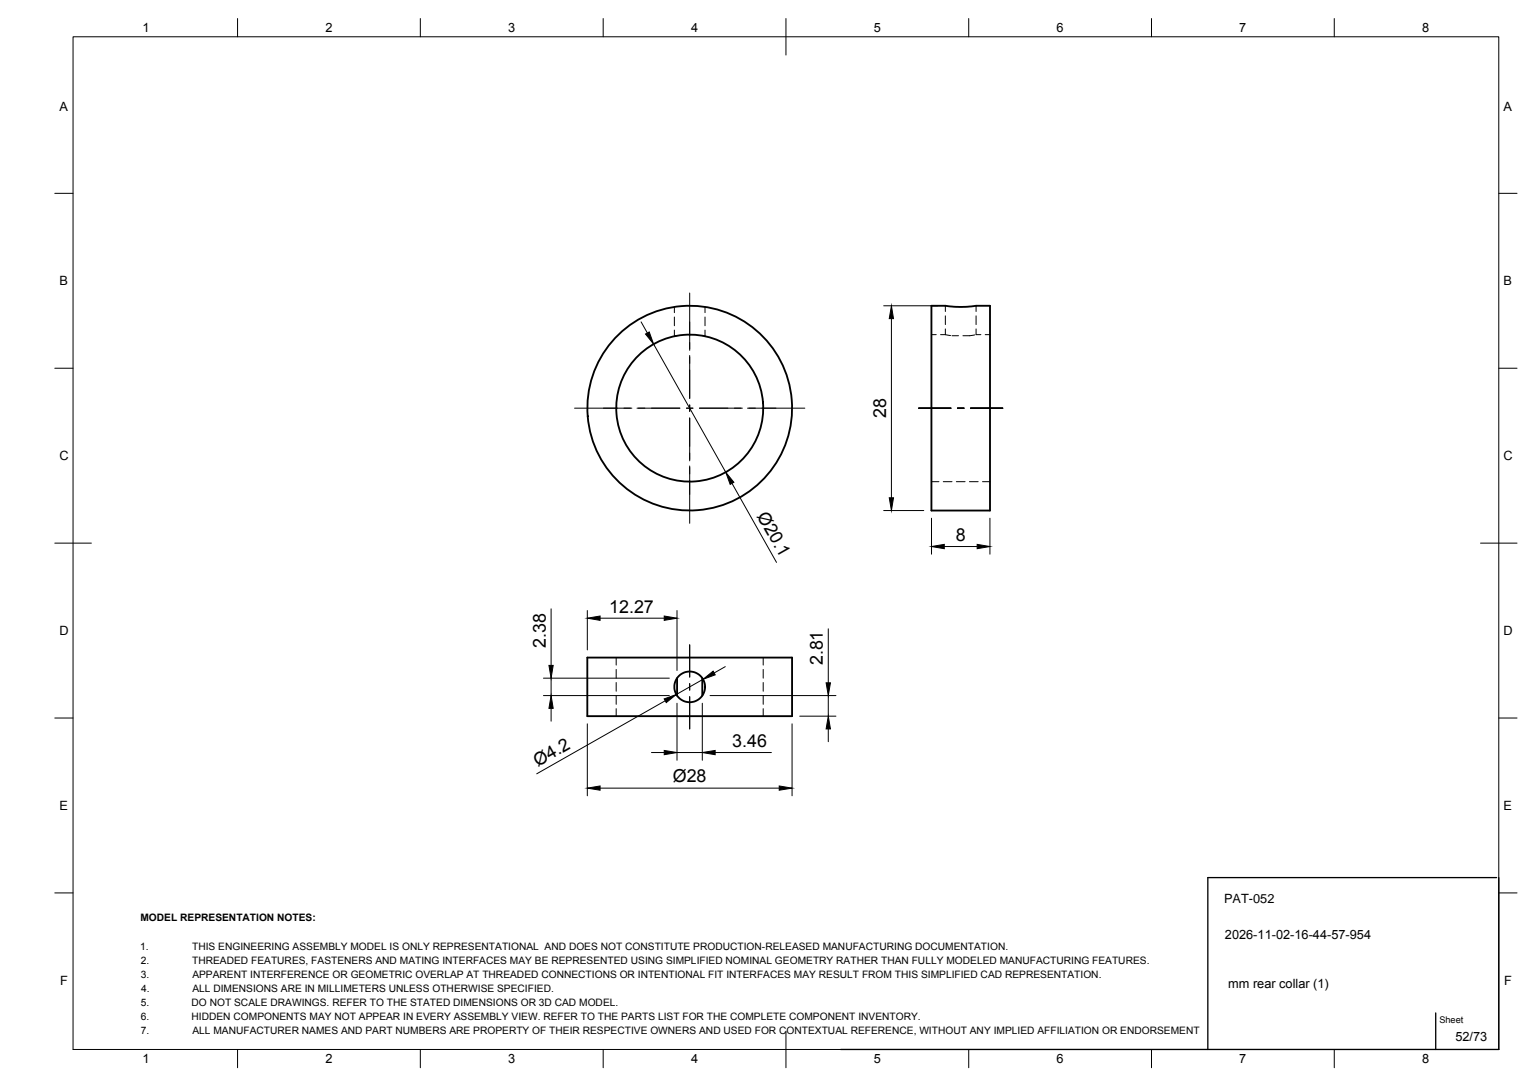
ISO-10303-21;
HEADER;
/* Generated by software containing ST-Developer
 * from STEP Tools, Inc. (www.steptools.com) 
 */

FILE_DESCRIPTION(
/* description */ ('Hand-crank gear train demonstrator'),
/* implementation_level */ '2;1');

FILE_NAME(
/* name */ 'mm rear collar (1).step',
/* time_stamp */ '2026-10-28T03:22:13-07:00',
/* author */ (''),
/* organization */ (''),
/* preprocessor_version */ 'ST-DEVELOPER v20.2',
/* originating_system */ 'Autodesk Translation Framework v15.17.0.0',
/* authorisation */ '');

FILE_SCHEMA (('AUTOMOTIVE_DESIGN { 1 0 10303 214 3 1 1 }'));
ENDSEC;

DATA;
#10=MECHANICAL_DESIGN_GEOMETRIC_PRESENTATION_REPRESENTATION('',(#1246),#62758);
#895=B_SPLINE_CURVE_WITH_KNOTS('',3,(#26487,#26488,#26489,#26490,#26491,
#26492,#26493,#26494,#26495,#26496,#26497,#26498,#26499,#26500),
 .UNSPECIFIED.,.F.,.F.,(4,2,2,2,2,2,4),(0.75600573798703,0.793568827564647,
0.872922520054202,0.952276212543757,1.03162990503331,1.11098359752287,1.14854668710048),
 .UNSPECIFIED.);
#896=B_SPLINE_CURVE_WITH_KNOTS('',3,(#26506,#26507,#26508,#26509,#26510,
#26511,#26512,#26513,#26514,#26515,#26516,#26517,#26518,#26519,#26520,#26521,
#26522,#26523),.UNSPECIFIED.,.F.,.F.,(4,2,2,2,2,2,2,2,4),(0.,0.0792334805614372,
0.158466961122874,0.237699060165217,0.31693115920756,0.396163258249903,
0.475395357292246,0.554628837853683,0.63386231841512),.UNSPECIFIED.);
#897=B_SPLINE_CURVE_WITH_KNOTS('',3,(#26524,#26525,#26526,#26527,#26528,
#26529,#26530,#26531,#26532,#26533,#26534,#26535,#26536,#26537,#26538,#26539,
#26540,#26541),.UNSPECIFIED.,.F.,.F.,(4,2,2,2,2,2,2,2,4),(0.63386231841512,
0.713095798976557,0.792329279537994,0.871561378580337,0.95079347762268,
1.03002557666502,1.10925767570737,1.1884911562688,1.26772463683024),
 .UNSPECIFIED.);
#898=B_SPLINE_CURVE_WITH_KNOTS('',3,(#26544,#26545,#26546,#26547,#26548,
#26549,#26550,#26551,#26552,#26553,#26554,#26555,#26556,#26557),
 .UNSPECIFIED.,.F.,.F.,(4,2,2,2,2,2,4),(0.121154929624526,0.158718019202142,
0.238071711691697,0.317425404181252,0.396779096670807,0.476132789160362,
0.513695878737979),.UNSPECIFIED.);
#1103=SHAPE_REPRESENTATION_RELATIONSHIP('SRR','None',#63079,#1167);
#1167=ADVANCED_BREP_SHAPE_REPRESENTATION('',(#1321),#62733);
#1246=STYLED_ITEM('',(#63448),#1321);
#1321=MANIFOLD_SOLID_BREP('Body1',#16430);
#1580=FACE_BOUND('',#3832,.T.);
#1581=FACE_BOUND('',#3834,.T.);
#1582=FACE_BOUND('',#3836,.T.);
#1583=FACE_BOUND('',#3838,.T.);
#1951=PLANE('',#18180);
#1952=PLANE('',#18185);
#1953=PLANE('',#18192);
#1954=PLANE('',#18193);
#2654=FACE_OUTER_BOUND('',#3828,.T.);
#2655=FACE_OUTER_BOUND('',#3829,.T.);
#2656=FACE_OUTER_BOUND('',#3830,.T.);
#2657=FACE_OUTER_BOUND('',#3831,.T.);
#2658=FACE_OUTER_BOUND('',#3833,.T.);
#2659=FACE_OUTER_BOUND('',#3835,.T.);
#2660=FACE_OUTER_BOUND('',#3837,.T.);
#3828=EDGE_LOOP('',(#13095,#13096));
#3829=EDGE_LOOP('',(#13097,#13098,#13099,#13100,#13101,#13102,#13103,#13104,
#13105));
#3830=EDGE_LOOP('',(#13106,#13107,#13108));
#3831=EDGE_LOOP('',(#13109,#13110,#13111,#13112));
#3832=EDGE_LOOP('',(#13113,#13114,#13115,#13116));
#3833=EDGE_LOOP('',(#13117,#13118,#13119,#13120));
#3834=EDGE_LOOP('',(#13121,#13122));
#3835=EDGE_LOOP('',(#13123));
#3836=EDGE_LOOP('',(#13124));
#3837=EDGE_LOOP('',(#13125));
#3838=EDGE_LOOP('',(#13126));
#4948=LINE('',#26483,#6080);
#4949=LINE('',#26504,#6081);
#4950=LINE('',#26559,#6082);
#4951=LINE('',#26564,#6083);
#4952=LINE('',#26570,#6084);
#6080=VECTOR('',#21539,1.);
#6081=VECTOR('',#21546,0.21);
#6082=VECTOR('',#21551,1.);
#6083=VECTOR('',#21556,1.005);
#6084=VECTOR('',#21563,1.4);
#6982=CIRCLE('',#18181,0.21);
#6983=CIRCLE('',#18183,0.21);
#6984=CIRCLE('',#18184,0.21);
#6985=CIRCLE('',#18187,1.005);
#6986=CIRCLE('',#18188,1.005);
#6987=CIRCLE('',#18190,1.4);
#6988=CIRCLE('',#18191,1.4);
#7979=VERTEX_POINT('',#26481);
#7980=VERTEX_POINT('',#26482);
#7981=VERTEX_POINT('',#26486);
#7982=VERTEX_POINT('',#26501);
#7983=VERTEX_POINT('',#26503);
#7984=VERTEX_POINT('',#26505);
#7985=VERTEX_POINT('',#26542);
#7986=VERTEX_POINT('',#26561);
#7987=VERTEX_POINT('',#26563);
#7988=VERTEX_POINT('',#26567);
#7989=VERTEX_POINT('',#26569);
#9799=EDGE_CURVE('',#7979,#7980,#4948,.T.);
#9800=EDGE_CURVE('',#7979,#7980,#6982,.T.);
#9801=EDGE_CURVE('',#7981,#7979,#895,.T.);
#9802=EDGE_CURVE('',#7982,#7981,#6983,.T.);
#9803=EDGE_CURVE('',#7982,#7983,#4949,.T.);
#9804=EDGE_CURVE('',#7984,#7983,#896,.T.);
#9805=EDGE_CURVE('',#7983,#7984,#897,.T.);
#9806=EDGE_CURVE('',#7985,#7982,#6984,.T.);
#9807=EDGE_CURVE('',#7980,#7985,#898,.T.);
#9808=EDGE_CURVE('',#7985,#7981,#4950,.T.);
#9809=EDGE_CURVE('',#7986,#7986,#6985,.T.);
#9810=EDGE_CURVE('',#7986,#7987,#4951,.T.);
#9811=EDGE_CURVE('',#7987,#7987,#6986,.T.);
#9812=EDGE_CURVE('',#7988,#7988,#6987,.T.);
#9813=EDGE_CURVE('',#7988,#7989,#4952,.T.);
#9814=EDGE_CURVE('',#7989,#7989,#6988,.T.);
#13095=ORIENTED_EDGE('',*,*,#9799,.F.);
#13096=ORIENTED_EDGE('',*,*,#9800,.T.);
#13097=ORIENTED_EDGE('',*,*,#9801,.F.);
#13098=ORIENTED_EDGE('',*,*,#9802,.F.);
#13099=ORIENTED_EDGE('',*,*,#9803,.T.);
#13100=ORIENTED_EDGE('',*,*,#9804,.F.);
#13101=ORIENTED_EDGE('',*,*,#9805,.F.);
#13102=ORIENTED_EDGE('',*,*,#9803,.F.);
#13103=ORIENTED_EDGE('',*,*,#9806,.F.);
#13104=ORIENTED_EDGE('',*,*,#9807,.F.);
#13105=ORIENTED_EDGE('',*,*,#9800,.F.);
#13106=ORIENTED_EDGE('',*,*,#9808,.F.);
#13107=ORIENTED_EDGE('',*,*,#9806,.T.);
#13108=ORIENTED_EDGE('',*,*,#9802,.T.);
#13109=ORIENTED_EDGE('',*,*,#9809,.F.);
#13110=ORIENTED_EDGE('',*,*,#9810,.T.);
#13111=ORIENTED_EDGE('',*,*,#9811,.T.);
#13112=ORIENTED_EDGE('',*,*,#9810,.F.);
#13113=ORIENTED_EDGE('',*,*,#9807,.T.);
#13114=ORIENTED_EDGE('',*,*,#9808,.T.);
#13115=ORIENTED_EDGE('',*,*,#9801,.T.);
#13116=ORIENTED_EDGE('',*,*,#9799,.T.);
#13117=ORIENTED_EDGE('',*,*,#9812,.F.);
#13118=ORIENTED_EDGE('',*,*,#9813,.T.);
#13119=ORIENTED_EDGE('',*,*,#9814,.T.);
#13120=ORIENTED_EDGE('',*,*,#9813,.F.);
#13121=ORIENTED_EDGE('',*,*,#9804,.T.);
#13122=ORIENTED_EDGE('',*,*,#9805,.T.);
#13123=ORIENTED_EDGE('',*,*,#9812,.T.);
#13124=ORIENTED_EDGE('',*,*,#9809,.T.);
#13125=ORIENTED_EDGE('',*,*,#9814,.F.);
#13126=ORIENTED_EDGE('',*,*,#9811,.F.);
#15326=CYLINDRICAL_SURFACE('',#18182,0.21);
#15327=CYLINDRICAL_SURFACE('',#18186,1.005);
#15328=CYLINDRICAL_SURFACE('',#18189,1.4);
#15964=ADVANCED_FACE('',(#2654),#1951,.T.);
#15965=ADVANCED_FACE('',(#2655),#15326,.F.);
#15966=ADVANCED_FACE('',(#2656),#1952,.T.);
#15967=ADVANCED_FACE('',(#2657,#1580),#15327,.F.);
#15968=ADVANCED_FACE('',(#2658,#1581),#15328,.T.);
#15969=ADVANCED_FACE('',(#2659,#1582),#1953,.T.);
#15970=ADVANCED_FACE('',(#2660,#1583),#1954,.F.);
#16430=CLOSED_SHELL('',(#15964,#15965,#15966,#15967,#15968,#15969,#15970));
#18179=AXIS2_PLACEMENT_3D('',#26479,#21535,#21536);
#18180=AXIS2_PLACEMENT_3D('',#26480,#21537,#21538);
#18181=AXIS2_PLACEMENT_3D('',#26484,#21540,#21541);
#18182=AXIS2_PLACEMENT_3D('',#26485,#21542,#21543);
#18183=AXIS2_PLACEMENT_3D('',#26502,#21544,#21545);
#18184=AXIS2_PLACEMENT_3D('',#26543,#21547,#21548);
#18185=AXIS2_PLACEMENT_3D('',#26558,#21549,#21550);
#18186=AXIS2_PLACEMENT_3D('',#26560,#21552,#21553);
#18187=AXIS2_PLACEMENT_3D('',#26562,#21554,#21555);
#18188=AXIS2_PLACEMENT_3D('',#26565,#21557,#21558);
#18189=AXIS2_PLACEMENT_3D('',#26566,#21559,#21560);
#18190=AXIS2_PLACEMENT_3D('',#26568,#21561,#21562);
#18191=AXIS2_PLACEMENT_3D('',#26571,#21564,#21565);
#18192=AXIS2_PLACEMENT_3D('',#26572,#21566,#21567);
#18193=AXIS2_PLACEMENT_3D('',#26573,#21568,#21569);
#21535=DIRECTION('axis',(0.,0.,1.));
#21536=DIRECTION('refdir',(1.,0.,0.));
#21537=DIRECTION('center_axis',(0.,0.,1.));
#21538=DIRECTION('ref_axis',(1.,0.,0.));
#21539=DIRECTION('',(0.,1.,0.));
#21540=DIRECTION('center_axis',(0.,0.,1.));
#21541=DIRECTION('ref_axis',(1.,0.,0.));
#21542=DIRECTION('center_axis',(0.,0.,1.));
#21543=DIRECTION('ref_axis',(1.,0.,0.));
#21544=DIRECTION('center_axis',(0.,0.,1.));
#21545=DIRECTION('ref_axis',(1.,0.,0.));
#21546=DIRECTION('',(0.,0.,1.));
#21547=DIRECTION('center_axis',(0.,0.,1.));
#21548=DIRECTION('ref_axis',(1.,0.,0.));
#21549=DIRECTION('center_axis',(0.,0.,1.));
#21550=DIRECTION('ref_axis',(1.,0.,0.));
#21551=DIRECTION('',(0.,-1.,0.));
#21552=DIRECTION('center_axis',(0.,1.,0.));
#21553=DIRECTION('ref_axis',(1.,0.,0.));
#21554=DIRECTION('center_axis',(0.,-1.,0.));
#21555=DIRECTION('ref_axis',(1.,0.,0.));
#21556=DIRECTION('',(0.,-1.,0.));
#21557=DIRECTION('center_axis',(0.,-1.,0.));
#21558=DIRECTION('ref_axis',(1.,0.,0.));
#21559=DIRECTION('center_axis',(0.,1.,0.));
#21560=DIRECTION('ref_axis',(1.,0.,0.));
#21561=DIRECTION('center_axis',(0.,1.,0.));
#21562=DIRECTION('ref_axis',(1.,0.,0.));
#21563=DIRECTION('',(0.,-1.,0.));
#21564=DIRECTION('center_axis',(0.,1.,0.));
#21565=DIRECTION('ref_axis',(1.,0.,0.));
#21566=DIRECTION('center_axis',(0.,1.,0.));
#21567=DIRECTION('ref_axis',(1.,0.,0.));
#21568=DIRECTION('center_axis',(0.,1.,0.));
#21569=DIRECTION('ref_axis',(1.,0.,0.));
#26479=CARTESIAN_POINT('',(0.,0.,0.));
#26480=CARTESIAN_POINT('Origin',(6.,-3.2,9.99));
#26481=CARTESIAN_POINT('',(6.17298843892005,-3.31905880899792,9.99));
#26482=CARTESIAN_POINT('',(6.17298843892005,-3.08094119100208,9.99));
#26483=CARTESIAN_POINT('',(6.17298843892005,-3.6,9.99));
#26484=CARTESIAN_POINT('Origin',(6.,-3.2,9.99));
#26485=CARTESIAN_POINT('Origin',(6.,-3.2,9.99));
#26486=CARTESIAN_POINT('',(5.82701156107995,-3.31905880899792,9.99));
#26487=CARTESIAN_POINT('Ctrl Pts',(5.82701156107995,-3.31905880899792,9.99));
#26488=CARTESIAN_POINT('Ctrl Pts',(5.83440513468869,-3.3298014223953,9.99129192197638));
#26489=CARTESIAN_POINT('Ctrl Pts',(5.8427028612744,-3.33968770937275,9.99265394943905));
#26490=CARTESIAN_POINT('Ctrl Pts',(5.87010792615492,-3.36709277425327,9.9967480843909));
#26491=CARTESIAN_POINT('Ctrl Pts',(5.89366983224072,-3.38324205633295,9.99969589327638));
#26492=CARTESIAN_POINT('Ctrl Pts',(5.94538709536759,-3.40469779396491,10.0038502947236));
#26493=CARTESIAN_POINT('Ctrl Pts',(5.97354876917015,-3.41,10.005));
#26494=CARTESIAN_POINT('Ctrl Pts',(6.02645123082985,-3.41,10.005));
#26495=CARTESIAN_POINT('Ctrl Pts',(6.05461290463241,-3.40469779396491,10.0038502947236));
#26496=CARTESIAN_POINT('Ctrl Pts',(6.10633016775928,-3.38324205633295,9.99969589327638));
#26497=CARTESIAN_POINT('Ctrl Pts',(6.12989207384508,-3.36709277425327,9.9967480843909));
#26498=CARTESIAN_POINT('Ctrl Pts',(6.1572971387256,-3.33968770937275,9.99265394943905));
#26499=CARTESIAN_POINT('Ctrl Pts',(6.16559486531131,-3.3298014223953,9.99129192197638));
#26500=CARTESIAN_POINT('Ctrl Pts',(6.17298843892005,-3.31905880899792,9.99));
#26501=CARTESIAN_POINT('',(5.79,-3.2,9.99));
#26502=CARTESIAN_POINT('Origin',(6.,-3.2,9.99));
#26503=CARTESIAN_POINT('',(5.79,-3.2,10.38416039533));
#26504=CARTESIAN_POINT('',(5.79,-3.2,9.99));
#26505=CARTESIAN_POINT('',(6.21,-3.2,10.38416039533));
#26506=CARTESIAN_POINT('Ctrl Pts',(6.21,-3.2,10.38416039533));
#26507=CARTESIAN_POINT('Ctrl Pts',(6.21,-3.22641116018715,10.38416039533));
#26508=CARTESIAN_POINT('Ctrl Pts',(6.20471354911189,-3.2545550596171,10.3849944296993));
#26509=CARTESIAN_POINT('Ctrl Pts',(6.18326999585849,-3.30628264999174,10.3879947099895));
#26510=CARTESIAN_POINT('Ctrl Pts',(6.16711503760643,-3.32986981049192,10.3901162943626));
#26511=CARTESIAN_POINT('Ctrl Pts',(6.12987013519678,-3.36711471290157,10.394089123191));
#26512=CARTESIAN_POINT('Ctrl Pts',(6.10628283459019,-3.38326992585508,10.3962002442067));
#26513=CARTESIAN_POINT('Ctrl Pts',(6.05455476560391,-3.40471366447292,10.3991765222353));
#26514=CARTESIAN_POINT('Ctrl Pts',(6.02641069968078,-3.41,10.4));
#26515=CARTESIAN_POINT('Ctrl Pts',(5.97358930031922,-3.41,10.4));
#26516=CARTESIAN_POINT('Ctrl Pts',(5.94544523439609,-3.40471366447292,10.3991765222353));
#26517=CARTESIAN_POINT('Ctrl Pts',(5.89371716540981,-3.38326992585508,10.3962002442067));
#26518=CARTESIAN_POINT('Ctrl Pts',(5.87012986480322,-3.36711471290157,10.394089123191));
#26519=CARTESIAN_POINT('Ctrl Pts',(5.83288496239357,-3.32986981049192,10.3901162943626));
#26520=CARTESIAN_POINT('Ctrl Pts',(5.81673000414151,-3.30628264999174,10.3879947099895));
#26521=CARTESIAN_POINT('Ctrl Pts',(5.79528645088811,-3.2545550596171,10.3849944296993));
#26522=CARTESIAN_POINT('Ctrl Pts',(5.79,-3.22641116018715,10.38416039533));
#26523=CARTESIAN_POINT('Ctrl Pts',(5.79,-3.2,10.38416039533));
#26524=CARTESIAN_POINT('Ctrl Pts',(5.79,-3.2,10.38416039533));
#26525=CARTESIAN_POINT('Ctrl Pts',(5.79,-3.17358883981285,10.38416039533));
#26526=CARTESIAN_POINT('Ctrl Pts',(5.79528645088811,-3.1454449403829,10.3849944296993));
#26527=CARTESIAN_POINT('Ctrl Pts',(5.81673000414151,-3.09371735000826,10.3879947099895));
#26528=CARTESIAN_POINT('Ctrl Pts',(5.83288496239357,-3.07013018950808,10.3901162943626));
#26529=CARTESIAN_POINT('Ctrl Pts',(5.87012986480322,-3.03288528709844,10.394089123191));
#26530=CARTESIAN_POINT('Ctrl Pts',(5.89371716540981,-3.01673007414492,10.3962002442067));
#26531=CARTESIAN_POINT('Ctrl Pts',(5.94544523439609,-2.99528633552708,10.3991765222353));
#26532=CARTESIAN_POINT('Ctrl Pts',(5.97358930031922,-2.99,10.4));
#26533=CARTESIAN_POINT('Ctrl Pts',(6.02641069968078,-2.99,10.4));
#26534=CARTESIAN_POINT('Ctrl Pts',(6.05455476560391,-2.99528633552708,10.3991765222353));
#26535=CARTESIAN_POINT('Ctrl Pts',(6.10628283459019,-3.01673007414492,10.3962002442067));
#26536=CARTESIAN_POINT('Ctrl Pts',(6.12987013519678,-3.03288528709844,10.394089123191));
#26537=CARTESIAN_POINT('Ctrl Pts',(6.16711503760643,-3.07013018950808,10.3901162943626));
#26538=CARTESIAN_POINT('Ctrl Pts',(6.18326999585849,-3.09371735000826,10.3879947099895));
#26539=CARTESIAN_POINT('Ctrl Pts',(6.20471354911189,-3.1454449403829,10.3849944296993));
#26540=CARTESIAN_POINT('Ctrl Pts',(6.21,-3.17358883981285,10.38416039533));
#26541=CARTESIAN_POINT('Ctrl Pts',(6.21,-3.2,10.38416039533));
#26542=CARTESIAN_POINT('',(5.82701156107995,-3.08094119100208,9.99));
#26543=CARTESIAN_POINT('Origin',(6.,-3.2,9.99));
#26544=CARTESIAN_POINT('Ctrl Pts',(6.17298843892005,-3.08094119100208,9.99));
#26545=CARTESIAN_POINT('Ctrl Pts',(6.16559486531131,-3.0701985776047,9.99129192197638));
#26546=CARTESIAN_POINT('Ctrl Pts',(6.15729713872561,-3.06031229062725,9.99265394943905));
#26547=CARTESIAN_POINT('Ctrl Pts',(6.12989207384508,-3.03290722574673,9.9967480843909));
#26548=CARTESIAN_POINT('Ctrl Pts',(6.10633016775929,-3.01675794366705,9.99969589327638));
#26549=CARTESIAN_POINT('Ctrl Pts',(6.05461290463241,-2.99530220603509,10.0038502947236));
#26550=CARTESIAN_POINT('Ctrl Pts',(6.02645123082985,-2.99,10.005));
#26551=CARTESIAN_POINT('Ctrl Pts',(5.97354876917015,-2.99,10.005));
#26552=CARTESIAN_POINT('Ctrl Pts',(5.94538709536759,-2.99530220603509,10.0038502947236));
#26553=CARTESIAN_POINT('Ctrl Pts',(5.89366983224072,-3.01675794366705,9.99969589327638));
#26554=CARTESIAN_POINT('Ctrl Pts',(5.87010792615492,-3.03290722574673,9.9967480843909));
#26555=CARTESIAN_POINT('Ctrl Pts',(5.8427028612744,-3.06031229062725,9.99265394943905));
#26556=CARTESIAN_POINT('Ctrl Pts',(5.83440513468869,-3.0701985776047,9.99129192197638));
#26557=CARTESIAN_POINT('Ctrl Pts',(5.82701156107995,-3.08094119100208,9.99));
#26558=CARTESIAN_POINT('Origin',(6.,-3.2,9.99));
#26559=CARTESIAN_POINT('',(5.82701156107995,-3.6,9.99));
#26560=CARTESIAN_POINT('Origin',(6.,-3.6,9.));
#26561=CARTESIAN_POINT('',(4.995,-2.8,9.));
#26562=CARTESIAN_POINT('Origin',(6.,-2.8,9.));
#26563=CARTESIAN_POINT('',(4.995,-3.6,9.));
#26564=CARTESIAN_POINT('',(4.995,-3.6,9.));
#26565=CARTESIAN_POINT('Origin',(6.,-3.6,9.));
#26566=CARTESIAN_POINT('Origin',(6.,-3.6,9.));
#26567=CARTESIAN_POINT('',(4.6,-2.8,9.));
#26568=CARTESIAN_POINT('Origin',(6.,-2.8,9.));
#26569=CARTESIAN_POINT('',(4.6,-3.6,9.));
#26570=CARTESIAN_POINT('',(4.6,-3.6,9.));
#26571=CARTESIAN_POINT('Origin',(6.,-3.6,9.));
#26572=CARTESIAN_POINT('Origin',(6.,-2.8,9.));
#26573=CARTESIAN_POINT('Origin',(6.,-3.6,9.));
#62659=UNCERTAINTY_MEASURE_WITH_UNIT(LENGTH_MEASURE(0.001),#62759,
'DISTANCE_ACCURACY_VALUE',
'Maximum model space distance between geometric entities at asserted c
onnectivities');
#62684=UNCERTAINTY_MEASURE_WITH_UNIT(LENGTH_MEASURE(0.001),#62759,
'DISTANCE_ACCURACY_VALUE',
'Maximum model space distance between geometric entities at asserted c
onnectivities');
#62733=(
GEOMETRIC_REPRESENTATION_CONTEXT(3)
GLOBAL_UNCERTAINTY_ASSIGNED_CONTEXT((#62659))
GLOBAL_UNIT_ASSIGNED_CONTEXT((#62759,#62761,#62762))
REPRESENTATION_CONTEXT('','3D')
);
#62758=(
GEOMETRIC_REPRESENTATION_CONTEXT(3)
GLOBAL_UNCERTAINTY_ASSIGNED_CONTEXT((#62684))
GLOBAL_UNIT_ASSIGNED_CONTEXT((#62759,#62761,#62762))
REPRESENTATION_CONTEXT('','3D')
);
#62759=(
LENGTH_UNIT()
NAMED_UNIT(*)
SI_UNIT(.CENTI.,.METRE.)
);
#62761=(
NAMED_UNIT(*)
PLANE_ANGLE_UNIT()
SI_UNIT($,.RADIAN.)
);
#62762=(
NAMED_UNIT(*)
SI_UNIT($,.STERADIAN.)
SOLID_ANGLE_UNIT()
);
#62811=SHAPE_DEFINITION_REPRESENTATION(#62894,#63079);
#62894=PRODUCT_DEFINITION_SHAPE('',$,#63153);
#63079=SHAPE_REPRESENTATION('',(#18179),#62733);
#63104=PRODUCT_DEFINITION_CONTEXT('part definition',#63325,'design');
#63153=PRODUCT_DEFINITION('mm rear collar (1)','mm rear collar (1)',#63226,
#63104);
#63226=PRODUCT_DEFINITION_FORMATION('',$,#63375);
#63325=APPLICATION_CONTEXT(
'Core Data for Automotive Mechanical Design Process');
#63326=PRODUCT_CONTEXT('part definition',#63325,'mechanical');
#63375=PRODUCT('mm rear collar (1)','mm rear collar (1)','mm rear collar (1)',
(#63326));
#63442=COLOUR_RGB('Light Blue',0.38,0.62,0.78);
#63443=FILL_AREA_STYLE_COLOUR('',#63442);
#63444=FILL_AREA_STYLE('',(#63443));
#63445=SURFACE_STYLE_FILL_AREA(#63444);
#63446=SURFACE_SIDE_STYLE('',(#63445));
#63447=SURFACE_STYLE_USAGE(.BOTH.,#63446);
#63448=PRESENTATION_STYLE_ASSIGNMENT((#63447));
ENDSEC;
END-ISO-10303-21;
